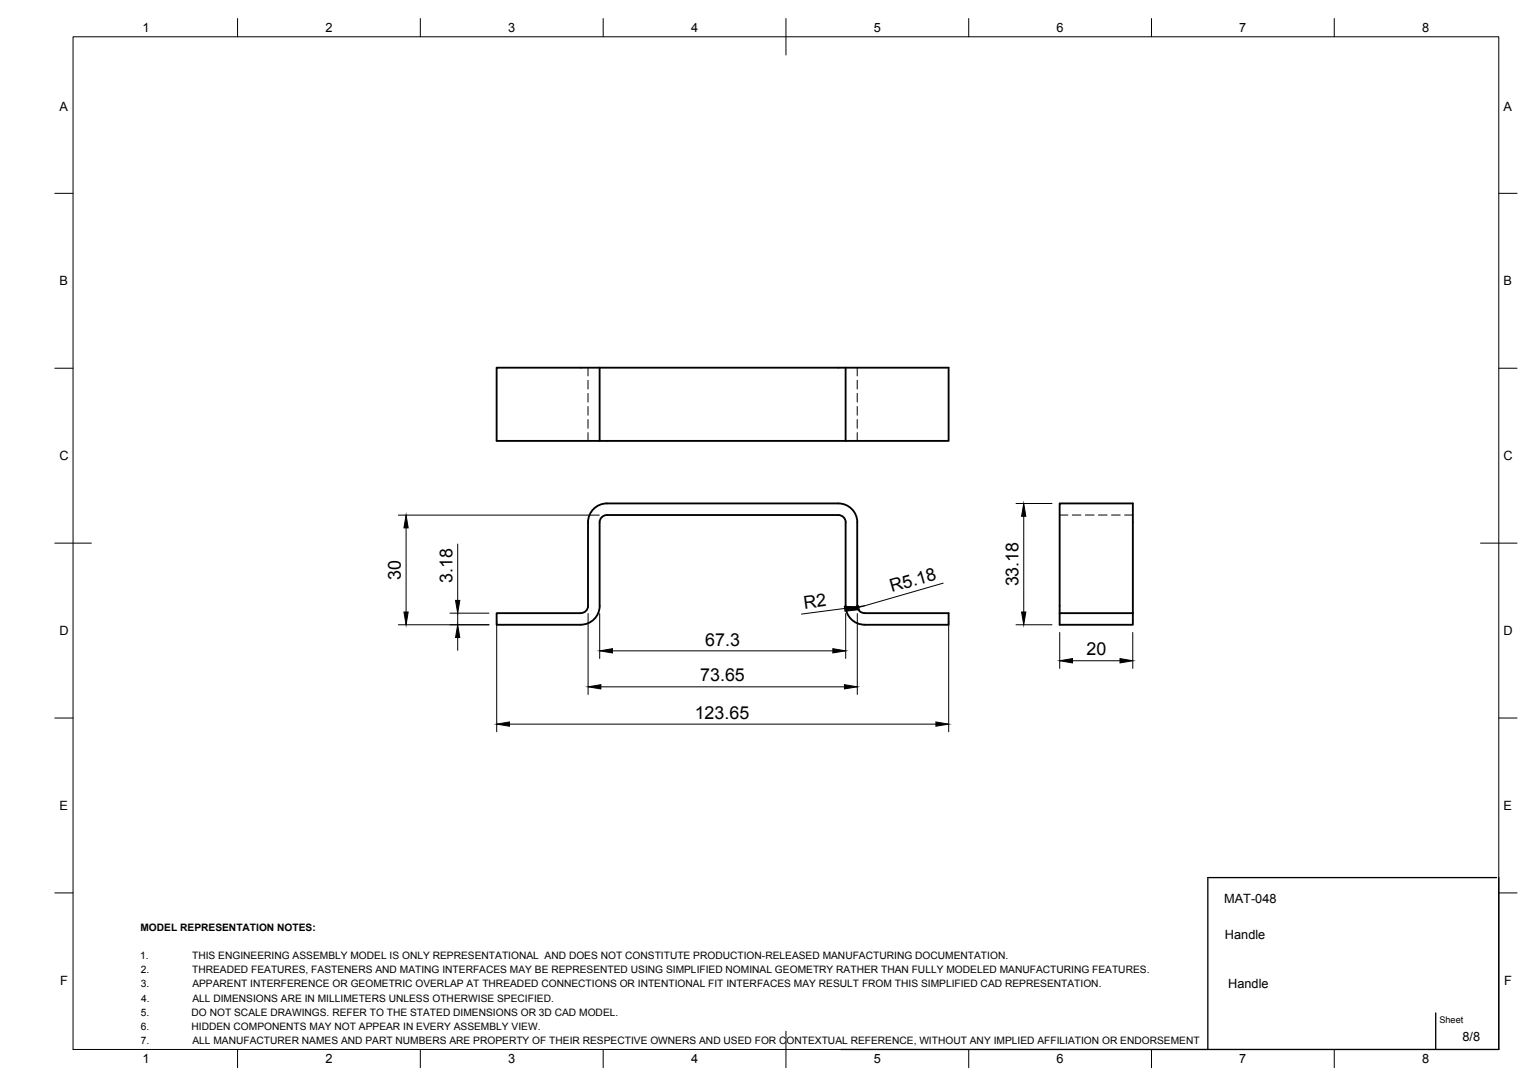
ISO-10303-21;
HEADER;
/* Generated by software containing ST-Developer
 * from STEP Tools, Inc. (www.steptools.com) 
 */

FILE_DESCRIPTION(
/* description */ ('STEP AP214'),
/* implementation_level */ '2;1');

FILE_NAME(
/* name */ 'Handle.step',
/* time_stamp */ '2026-11-14T22:24:45-08:00',
/* author */ (''),
/* organization */ (''),
/* preprocessor_version */ 'ST-DEVELOPER v20.2',
/* originating_system */ 'Autodesk Translation Framework v15.17.0.0',
/* authorisation */ '');

FILE_SCHEMA (('AUTOMOTIVE_DESIGN { 1 0 10303 214 3 1 1 }'));
ENDSEC;

DATA;
#10=MECHANICAL_DESIGN_GEOMETRIC_PRESENTATION_REPRESENTATION('',(#126),#5599);
#114=SHAPE_REPRESENTATION_RELATIONSHIP('SRR','None',#5642,#120);
#120=ADVANCED_BREP_SHAPE_REPRESENTATION('',(#132),#5594);
#126=STYLED_ITEM('',(#5681),#132);
#132=MANIFOLD_SOLID_BREP('Body1',#3308);
#157=CYLINDRICAL_SURFACE('',#3508,2.);
#158=CYLINDRICAL_SURFACE('',#3510,5.175);
#159=CYLINDRICAL_SURFACE('',#3512,5.175);
#160=CYLINDRICAL_SURFACE('',#3514,2.);
#161=CYLINDRICAL_SURFACE('',#3518,5.175);
#162=CYLINDRICAL_SURFACE('',#3520,2.);
#163=CYLINDRICAL_SURFACE('',#3522,2.);
#164=CYLINDRICAL_SURFACE('',#3524,5.175);
#209=CIRCLE('',#3474,2.);
#210=CIRCLE('',#3475,5.175);
#211=CIRCLE('',#3478,2.);
#212=CIRCLE('',#3479,5.175);
#213=CIRCLE('',#3482,5.175);
#214=CIRCLE('',#3483,2.);
#215=CIRCLE('',#3486,5.175);
#216=CIRCLE('',#3487,2.);
#217=CIRCLE('',#3490,5.175);
#218=CIRCLE('',#3491,2.);
#219=CIRCLE('',#3494,5.175);
#220=CIRCLE('',#3495,2.);
#221=CIRCLE('',#3498,2.);
#222=CIRCLE('',#3499,5.175);
#223=CIRCLE('',#3502,2.);
#224=CIRCLE('',#3503,5.175);
#347=FACE_OUTER_BOUND('',#523,.T.);
#348=FACE_OUTER_BOUND('',#524,.T.);
#349=FACE_OUTER_BOUND('',#525,.T.);
#350=FACE_OUTER_BOUND('',#526,.T.);
#351=FACE_OUTER_BOUND('',#527,.T.);
#352=FACE_OUTER_BOUND('',#528,.T.);
#353=FACE_OUTER_BOUND('',#529,.T.);
#354=FACE_OUTER_BOUND('',#530,.T.);
#355=FACE_OUTER_BOUND('',#531,.T.);
#356=FACE_OUTER_BOUND('',#532,.T.);
#357=FACE_OUTER_BOUND('',#533,.T.);
#358=FACE_OUTER_BOUND('',#534,.T.);
#359=FACE_OUTER_BOUND('',#535,.T.);
#360=FACE_OUTER_BOUND('',#536,.T.);
#361=FACE_OUTER_BOUND('',#537,.T.);
#362=FACE_OUTER_BOUND('',#538,.T.);
#363=FACE_OUTER_BOUND('',#539,.T.);
#364=FACE_OUTER_BOUND('',#540,.T.);
#365=FACE_OUTER_BOUND('',#541,.T.);
#366=FACE_OUTER_BOUND('',#542,.T.);
#367=FACE_OUTER_BOUND('',#543,.T.);
#368=FACE_OUTER_BOUND('',#544,.T.);
#369=FACE_OUTER_BOUND('',#545,.T.);
#370=FACE_OUTER_BOUND('',#546,.T.);
#371=FACE_OUTER_BOUND('',#547,.T.);
#372=FACE_OUTER_BOUND('',#548,.T.);
#373=FACE_OUTER_BOUND('',#549,.T.);
#374=FACE_OUTER_BOUND('',#550,.T.);
#375=FACE_OUTER_BOUND('',#551,.T.);
#376=FACE_OUTER_BOUND('',#552,.T.);
#377=FACE_OUTER_BOUND('',#553,.T.);
#378=FACE_OUTER_BOUND('',#554,.T.);
#379=FACE_OUTER_BOUND('',#555,.T.);
#380=FACE_OUTER_BOUND('',#556,.T.);
#381=FACE_OUTER_BOUND('',#557,.T.);
#382=FACE_OUTER_BOUND('',#558,.T.);
#383=FACE_OUTER_BOUND('',#559,.T.);
#384=FACE_OUTER_BOUND('',#560,.T.);
#523=EDGE_LOOP('',(#2483,#2484,#2485,#2486));
#524=EDGE_LOOP('',(#2487,#2488,#2489,#2490));
#525=EDGE_LOOP('',(#2491,#2492,#2493,#2494));
#526=EDGE_LOOP('',(#2495,#2496,#2497,#2498));
#527=EDGE_LOOP('',(#2499,#2500,#2501,#2502));
#528=EDGE_LOOP('',(#2503,#2504,#2505,#2506));
#529=EDGE_LOOP('',(#2507,#2508,#2509,#2510));
#530=EDGE_LOOP('',(#2511,#2512,#2513,#2514));
#531=EDGE_LOOP('',(#2515,#2516,#2517,#2518));
#532=EDGE_LOOP('',(#2519,#2520,#2521,#2522));
#533=EDGE_LOOP('',(#2523,#2524,#2525,#2526));
#534=EDGE_LOOP('',(#2527,#2528,#2529,#2530));
#535=EDGE_LOOP('',(#2531,#2532,#2533,#2534));
#536=EDGE_LOOP('',(#2535,#2536,#2537,#2538));
#537=EDGE_LOOP('',(#2539,#2540,#2541,#2542));
#538=EDGE_LOOP('',(#2543,#2544,#2545,#2546));
#539=EDGE_LOOP('',(#2547,#2548,#2549,#2550));
#540=EDGE_LOOP('',(#2551,#2552,#2553,#2554));
#541=EDGE_LOOP('',(#2555,#2556,#2557,#2558));
#542=EDGE_LOOP('',(#2559,#2560,#2561,#2562));
#543=EDGE_LOOP('',(#2563,#2564,#2565,#2566));
#544=EDGE_LOOP('',(#2567,#2568,#2569,#2570));
#545=EDGE_LOOP('',(#2571,#2572,#2573,#2574));
#546=EDGE_LOOP('',(#2575,#2576,#2577,#2578));
#547=EDGE_LOOP('',(#2579,#2580,#2581,#2582));
#548=EDGE_LOOP('',(#2583,#2584,#2585,#2586));
#549=EDGE_LOOP('',(#2587,#2588,#2589,#2590));
#550=EDGE_LOOP('',(#2591,#2592,#2593,#2594));
#551=EDGE_LOOP('',(#2595,#2596,#2597,#2598));
#552=EDGE_LOOP('',(#2599,#2600,#2601,#2602));
#553=EDGE_LOOP('',(#2603,#2604,#2605,#2606));
#554=EDGE_LOOP('',(#2607,#2608,#2609,#2610));
#555=EDGE_LOOP('',(#2611,#2612,#2613,#2614));
#556=EDGE_LOOP('',(#2615,#2616,#2617,#2618));
#557=EDGE_LOOP('',(#2619,#2620,#2621,#2622));
#558=EDGE_LOOP('',(#2623,#2624,#2625,#2626));
#559=EDGE_LOOP('',(#2627,#2628,#2629,#2630));
#560=EDGE_LOOP('',(#2631,#2632,#2633,#2634));
#815=LINE('',#5031,#1171);
#816=LINE('',#5035,#1172);
#817=LINE('',#5039,#1173);
#818=LINE('',#5041,#1174);
#819=LINE('',#5042,#1175);
#820=LINE('',#5046,#1176);
#821=LINE('',#5050,#1177);
#822=LINE('',#5054,#1178);
#823=LINE('',#5056,#1179);
#824=LINE('',#5057,#1180);
#825=LINE('',#5061,#1181);
#826=LINE('',#5066,#1182);
#827=LINE('',#5068,#1183);
#828=LINE('',#5069,#1184);
#829=LINE('',#5073,#1185);
#830=LINE('',#5077,#1186);
#831=LINE('',#5080,#1187);
#832=LINE('',#5081,#1188);
#833=LINE('',#5085,#1189);
#834=LINE('',#5090,#1190);
#835=LINE('',#5092,#1191);
#836=LINE('',#5093,#1192);
#837=LINE('',#5097,#1193);
#838=LINE('',#5101,#1194);
#839=LINE('',#5104,#1195);
#840=LINE('',#5105,#1196);
#841=LINE('',#5109,#1197);
#842=LINE('',#5114,#1198);
#843=LINE('',#5116,#1199);
#844=LINE('',#5117,#1200);
#845=LINE('',#5121,#1201);
#846=LINE('',#5125,#1202);
#847=LINE('',#5128,#1203);
#848=LINE('',#5129,#1204);
#849=LINE('',#5132,#1205);
#850=LINE('',#5133,#1206);
#851=LINE('',#5134,#1207);
#852=LINE('',#5137,#1208);
#853=LINE('',#5138,#1209);
#854=LINE('',#5140,#1210);
#855=LINE('',#5141,#1211);
#856=LINE('',#5143,#1212);
#857=LINE('',#5145,#1213);
#858=LINE('',#5147,#1214);
#859=LINE('',#5149,#1215);
#860=LINE('',#5151,#1216);
#861=LINE('',#5153,#1217);
#862=LINE('',#5155,#1218);
#863=LINE('',#5158,#1219);
#864=LINE('',#5159,#1220);
#865=LINE('',#5162,#1221);
#866=LINE('',#5163,#1222);
#867=LINE('',#5165,#1223);
#868=LINE('',#5166,#1224);
#869=LINE('',#5168,#1225);
#870=LINE('',#5170,#1226);
#871=LINE('',#5172,#1227);
#872=LINE('',#5174,#1228);
#873=LINE('',#5176,#1229);
#874=LINE('',#5178,#1230);
#1171=VECTOR('',#4037,1000.);
#1172=VECTOR('',#4040,1000.);
#1173=VECTOR('',#4045,1000.);
#1174=VECTOR('',#4046,1000.);
#1175=VECTOR('',#4047,1000.);
#1176=VECTOR('',#4050,1000.);
#1177=VECTOR('',#4053,1000.);
#1178=VECTOR('',#4058,1000.);
#1179=VECTOR('',#4059,1000.);
#1180=VECTOR('',#4060,1000.);
#1181=VECTOR('',#4063,1000.);
#1182=VECTOR('',#4070,1000.);
#1183=VECTOR('',#4071,1000.);
#1184=VECTOR('',#4072,1000.);
#1185=VECTOR('',#4075,1000.);
#1186=VECTOR('',#4078,1000.);
#1187=VECTOR('',#4083,1000.);
#1188=VECTOR('',#4084,1000.);
#1189=VECTOR('',#4087,1000.);
#1190=VECTOR('',#4094,1000.);
#1191=VECTOR('',#4095,1000.);
#1192=VECTOR('',#4096,1000.);
#1193=VECTOR('',#4099,1000.);
#1194=VECTOR('',#4102,1000.);
#1195=VECTOR('',#4107,1000.);
#1196=VECTOR('',#4108,1000.);
#1197=VECTOR('',#4111,1000.);
#1198=VECTOR('',#4118,1000.);
#1199=VECTOR('',#4119,1000.);
#1200=VECTOR('',#4120,1000.);
#1201=VECTOR('',#4123,1000.);
#1202=VECTOR('',#4126,1000.);
#1203=VECTOR('',#4131,1000.);
#1204=VECTOR('',#4132,1000.);
#1205=VECTOR('',#4135,1000.);
#1206=VECTOR('',#4136,1000.);
#1207=VECTOR('',#4137,1000.);
#1208=VECTOR('',#4140,1000.);
#1209=VECTOR('',#4141,1000.);
#1210=VECTOR('',#4144,1000.);
#1211=VECTOR('',#4145,1000.);
#1212=VECTOR('',#4148,1000.);
#1213=VECTOR('',#4151,1000.);
#1214=VECTOR('',#4154,1000.);
#1215=VECTOR('',#4157,1000.);
#1216=VECTOR('',#4160,1000.);
#1217=VECTOR('',#4163,1000.);
#1218=VECTOR('',#4166,1000.);
#1219=VECTOR('',#4169,1000.);
#1220=VECTOR('',#4170,1000.);
#1221=VECTOR('',#4173,1000.);
#1222=VECTOR('',#4174,1000.);
#1223=VECTOR('',#4177,1000.);
#1224=VECTOR('',#4178,1000.);
#1225=VECTOR('',#4181,1000.);
#1226=VECTOR('',#4184,1000.);
#1227=VECTOR('',#4187,1000.);
#1228=VECTOR('',#4190,1000.);
#1229=VECTOR('',#4193,1000.);
#1230=VECTOR('',#4196,1000.);
#1487=VERTEX_POINT('',#5029);
#1488=VERTEX_POINT('',#5030);
#1489=VERTEX_POINT('',#5032);
#1490=VERTEX_POINT('',#5034);
#1491=VERTEX_POINT('',#5038);
#1492=VERTEX_POINT('',#5040);
#1493=VERTEX_POINT('',#5044);
#1494=VERTEX_POINT('',#5045);
#1495=VERTEX_POINT('',#5047);
#1496=VERTEX_POINT('',#5049);
#1497=VERTEX_POINT('',#5053);
#1498=VERTEX_POINT('',#5055);
#1499=VERTEX_POINT('',#5059);
#1500=VERTEX_POINT('',#5060);
#1501=VERTEX_POINT('',#5065);
#1502=VERTEX_POINT('',#5067);
#1503=VERTEX_POINT('',#5071);
#1504=VERTEX_POINT('',#5072);
#1505=VERTEX_POINT('',#5074);
#1506=VERTEX_POINT('',#5076);
#1507=VERTEX_POINT('',#5083);
#1508=VERTEX_POINT('',#5084);
#1509=VERTEX_POINT('',#5089);
#1510=VERTEX_POINT('',#5091);
#1511=VERTEX_POINT('',#5095);
#1512=VERTEX_POINT('',#5096);
#1513=VERTEX_POINT('',#5098);
#1514=VERTEX_POINT('',#5100);
#1515=VERTEX_POINT('',#5107);
#1516=VERTEX_POINT('',#5108);
#1517=VERTEX_POINT('',#5113);
#1518=VERTEX_POINT('',#5115);
#1519=VERTEX_POINT('',#5119);
#1520=VERTEX_POINT('',#5120);
#1521=VERTEX_POINT('',#5122);
#1522=VERTEX_POINT('',#5124);
#1523=VERTEX_POINT('',#5131);
#1524=VERTEX_POINT('',#5136);
#1525=VERTEX_POINT('',#5157);
#1526=VERTEX_POINT('',#5161);
#1839=EDGE_CURVE('',#1487,#1488,#815,.T.);
#1840=EDGE_CURVE('',#1489,#1487,#209,.T.);
#1841=EDGE_CURVE('',#1490,#1489,#816,.T.);
#1842=EDGE_CURVE('',#1490,#1488,#210,.T.);
#1843=EDGE_CURVE('',#1487,#1491,#817,.T.);
#1844=EDGE_CURVE('',#1488,#1492,#818,.T.);
#1845=EDGE_CURVE('',#1492,#1491,#819,.T.);
#1846=EDGE_CURVE('',#1493,#1494,#820,.T.);
#1847=EDGE_CURVE('',#1493,#1495,#211,.T.);
#1848=EDGE_CURVE('',#1496,#1495,#821,.T.);
#1849=EDGE_CURVE('',#1494,#1496,#212,.T.);
#1850=EDGE_CURVE('',#1497,#1493,#822,.T.);
#1851=EDGE_CURVE('',#1498,#1494,#823,.T.);
#1852=EDGE_CURVE('',#1498,#1497,#824,.T.);
#1853=EDGE_CURVE('',#1499,#1500,#825,.T.);
#1854=EDGE_CURVE('',#1491,#1499,#213,.T.);
#1855=EDGE_CURVE('',#1492,#1500,#214,.T.);
#1856=EDGE_CURVE('',#1499,#1501,#826,.T.);
#1857=EDGE_CURVE('',#1500,#1502,#827,.T.);
#1858=EDGE_CURVE('',#1502,#1501,#828,.T.);
#1859=EDGE_CURVE('',#1503,#1504,#829,.T.);
#1860=EDGE_CURVE('',#1503,#1505,#215,.T.);
#1861=EDGE_CURVE('',#1506,#1505,#830,.T.);
#1862=EDGE_CURVE('',#1504,#1506,#216,.T.);
#1863=EDGE_CURVE('',#1495,#1503,#831,.T.);
#1864=EDGE_CURVE('',#1496,#1504,#832,.T.);
#1865=EDGE_CURVE('',#1507,#1508,#833,.T.);
#1866=EDGE_CURVE('',#1501,#1507,#217,.T.);
#1867=EDGE_CURVE('',#1502,#1508,#218,.T.);
#1868=EDGE_CURVE('',#1507,#1509,#834,.T.);
#1869=EDGE_CURVE('',#1508,#1510,#835,.T.);
#1870=EDGE_CURVE('',#1510,#1509,#836,.T.);
#1871=EDGE_CURVE('',#1511,#1512,#837,.T.);
#1872=EDGE_CURVE('',#1511,#1513,#219,.T.);
#1873=EDGE_CURVE('',#1514,#1513,#838,.T.);
#1874=EDGE_CURVE('',#1512,#1514,#220,.T.);
#1875=EDGE_CURVE('',#1505,#1511,#839,.T.);
#1876=EDGE_CURVE('',#1506,#1512,#840,.T.);
#1877=EDGE_CURVE('',#1515,#1516,#841,.T.);
#1878=EDGE_CURVE('',#1509,#1515,#221,.T.);
#1879=EDGE_CURVE('',#1510,#1516,#222,.T.);
#1880=EDGE_CURVE('',#1515,#1517,#842,.T.);
#1881=EDGE_CURVE('',#1516,#1518,#843,.T.);
#1882=EDGE_CURVE('',#1517,#1518,#844,.T.);
#1883=EDGE_CURVE('',#1519,#1520,#845,.T.);
#1884=EDGE_CURVE('',#1519,#1521,#223,.T.);
#1885=EDGE_CURVE('',#1522,#1521,#846,.T.);
#1886=EDGE_CURVE('',#1520,#1522,#224,.T.);
#1887=EDGE_CURVE('',#1513,#1519,#847,.T.);
#1888=EDGE_CURVE('',#1514,#1520,#848,.T.);
#1889=EDGE_CURVE('',#1522,#1523,#849,.T.);
#1890=EDGE_CURVE('',#1518,#1523,#850,.T.);
#1891=EDGE_CURVE('',#1516,#1522,#851,.T.);
#1892=EDGE_CURVE('',#1524,#1523,#852,.T.);
#1893=EDGE_CURVE('',#1517,#1524,#853,.T.);
#1894=EDGE_CURVE('',#1521,#1524,#854,.T.);
#1895=EDGE_CURVE('',#1515,#1521,#855,.T.);
#1896=EDGE_CURVE('',#1509,#1519,#856,.T.);
#1897=EDGE_CURVE('',#1507,#1513,#857,.T.);
#1898=EDGE_CURVE('',#1501,#1511,#858,.T.);
#1899=EDGE_CURVE('',#1499,#1505,#859,.T.);
#1900=EDGE_CURVE('',#1491,#1503,#860,.T.);
#1901=EDGE_CURVE('',#1487,#1495,#861,.T.);
#1902=EDGE_CURVE('',#1489,#1493,#862,.T.);
#1903=EDGE_CURVE('',#1525,#1497,#863,.T.);
#1904=EDGE_CURVE('',#1525,#1489,#864,.T.);
#1905=EDGE_CURVE('',#1526,#1498,#865,.T.);
#1906=EDGE_CURVE('',#1526,#1525,#866,.T.);
#1907=EDGE_CURVE('',#1490,#1494,#867,.T.);
#1908=EDGE_CURVE('',#1526,#1490,#868,.T.);
#1909=EDGE_CURVE('',#1488,#1496,#869,.T.);
#1910=EDGE_CURVE('',#1492,#1504,#870,.T.);
#1911=EDGE_CURVE('',#1500,#1506,#871,.T.);
#1912=EDGE_CURVE('',#1502,#1512,#872,.T.);
#1913=EDGE_CURVE('',#1508,#1514,#873,.T.);
#1914=EDGE_CURVE('',#1510,#1520,#874,.T.);
#2483=ORIENTED_EDGE('',*,*,#1839,.F.);
#2484=ORIENTED_EDGE('',*,*,#1840,.F.);
#2485=ORIENTED_EDGE('',*,*,#1841,.F.);
#2486=ORIENTED_EDGE('',*,*,#1842,.T.);
#2487=ORIENTED_EDGE('',*,*,#1843,.F.);
#2488=ORIENTED_EDGE('',*,*,#1839,.T.);
#2489=ORIENTED_EDGE('',*,*,#1844,.T.);
#2490=ORIENTED_EDGE('',*,*,#1845,.T.);
#2491=ORIENTED_EDGE('',*,*,#1846,.F.);
#2492=ORIENTED_EDGE('',*,*,#1847,.T.);
#2493=ORIENTED_EDGE('',*,*,#1848,.F.);
#2494=ORIENTED_EDGE('',*,*,#1849,.F.);
#2495=ORIENTED_EDGE('',*,*,#1850,.T.);
#2496=ORIENTED_EDGE('',*,*,#1846,.T.);
#2497=ORIENTED_EDGE('',*,*,#1851,.F.);
#2498=ORIENTED_EDGE('',*,*,#1852,.T.);
#2499=ORIENTED_EDGE('',*,*,#1853,.F.);
#2500=ORIENTED_EDGE('',*,*,#1854,.F.);
#2501=ORIENTED_EDGE('',*,*,#1845,.F.);
#2502=ORIENTED_EDGE('',*,*,#1855,.T.);
#2503=ORIENTED_EDGE('',*,*,#1856,.F.);
#2504=ORIENTED_EDGE('',*,*,#1853,.T.);
#2505=ORIENTED_EDGE('',*,*,#1857,.T.);
#2506=ORIENTED_EDGE('',*,*,#1858,.T.);
#2507=ORIENTED_EDGE('',*,*,#1859,.F.);
#2508=ORIENTED_EDGE('',*,*,#1860,.T.);
#2509=ORIENTED_EDGE('',*,*,#1861,.F.);
#2510=ORIENTED_EDGE('',*,*,#1862,.F.);
#2511=ORIENTED_EDGE('',*,*,#1863,.T.);
#2512=ORIENTED_EDGE('',*,*,#1859,.T.);
#2513=ORIENTED_EDGE('',*,*,#1864,.F.);
#2514=ORIENTED_EDGE('',*,*,#1848,.T.);
#2515=ORIENTED_EDGE('',*,*,#1865,.F.);
#2516=ORIENTED_EDGE('',*,*,#1866,.F.);
#2517=ORIENTED_EDGE('',*,*,#1858,.F.);
#2518=ORIENTED_EDGE('',*,*,#1867,.T.);
#2519=ORIENTED_EDGE('',*,*,#1868,.F.);
#2520=ORIENTED_EDGE('',*,*,#1865,.T.);
#2521=ORIENTED_EDGE('',*,*,#1869,.T.);
#2522=ORIENTED_EDGE('',*,*,#1870,.T.);
#2523=ORIENTED_EDGE('',*,*,#1871,.F.);
#2524=ORIENTED_EDGE('',*,*,#1872,.T.);
#2525=ORIENTED_EDGE('',*,*,#1873,.F.);
#2526=ORIENTED_EDGE('',*,*,#1874,.F.);
#2527=ORIENTED_EDGE('',*,*,#1875,.T.);
#2528=ORIENTED_EDGE('',*,*,#1871,.T.);
#2529=ORIENTED_EDGE('',*,*,#1876,.F.);
#2530=ORIENTED_EDGE('',*,*,#1861,.T.);
#2531=ORIENTED_EDGE('',*,*,#1877,.F.);
#2532=ORIENTED_EDGE('',*,*,#1878,.F.);
#2533=ORIENTED_EDGE('',*,*,#1870,.F.);
#2534=ORIENTED_EDGE('',*,*,#1879,.T.);
#2535=ORIENTED_EDGE('',*,*,#1880,.F.);
#2536=ORIENTED_EDGE('',*,*,#1877,.T.);
#2537=ORIENTED_EDGE('',*,*,#1881,.T.);
#2538=ORIENTED_EDGE('',*,*,#1882,.F.);
#2539=ORIENTED_EDGE('',*,*,#1883,.F.);
#2540=ORIENTED_EDGE('',*,*,#1884,.T.);
#2541=ORIENTED_EDGE('',*,*,#1885,.F.);
#2542=ORIENTED_EDGE('',*,*,#1886,.F.);
#2543=ORIENTED_EDGE('',*,*,#1887,.T.);
#2544=ORIENTED_EDGE('',*,*,#1883,.T.);
#2545=ORIENTED_EDGE('',*,*,#1888,.F.);
#2546=ORIENTED_EDGE('',*,*,#1873,.T.);
#2547=ORIENTED_EDGE('',*,*,#1889,.T.);
#2548=ORIENTED_EDGE('',*,*,#1890,.F.);
#2549=ORIENTED_EDGE('',*,*,#1881,.F.);
#2550=ORIENTED_EDGE('',*,*,#1891,.T.);
#2551=ORIENTED_EDGE('',*,*,#1892,.F.);
#2552=ORIENTED_EDGE('',*,*,#1893,.F.);
#2553=ORIENTED_EDGE('',*,*,#1882,.T.);
#2554=ORIENTED_EDGE('',*,*,#1890,.T.);
#2555=ORIENTED_EDGE('',*,*,#1894,.F.);
#2556=ORIENTED_EDGE('',*,*,#1895,.F.);
#2557=ORIENTED_EDGE('',*,*,#1880,.T.);
#2558=ORIENTED_EDGE('',*,*,#1893,.T.);
#2559=ORIENTED_EDGE('',*,*,#1884,.F.);
#2560=ORIENTED_EDGE('',*,*,#1896,.F.);
#2561=ORIENTED_EDGE('',*,*,#1878,.T.);
#2562=ORIENTED_EDGE('',*,*,#1895,.T.);
#2563=ORIENTED_EDGE('',*,*,#1887,.F.);
#2564=ORIENTED_EDGE('',*,*,#1897,.F.);
#2565=ORIENTED_EDGE('',*,*,#1868,.T.);
#2566=ORIENTED_EDGE('',*,*,#1896,.T.);
#2567=ORIENTED_EDGE('',*,*,#1872,.F.);
#2568=ORIENTED_EDGE('',*,*,#1898,.F.);
#2569=ORIENTED_EDGE('',*,*,#1866,.T.);
#2570=ORIENTED_EDGE('',*,*,#1897,.T.);
#2571=ORIENTED_EDGE('',*,*,#1875,.F.);
#2572=ORIENTED_EDGE('',*,*,#1899,.F.);
#2573=ORIENTED_EDGE('',*,*,#1856,.T.);
#2574=ORIENTED_EDGE('',*,*,#1898,.T.);
#2575=ORIENTED_EDGE('',*,*,#1860,.F.);
#2576=ORIENTED_EDGE('',*,*,#1900,.F.);
#2577=ORIENTED_EDGE('',*,*,#1854,.T.);
#2578=ORIENTED_EDGE('',*,*,#1899,.T.);
#2579=ORIENTED_EDGE('',*,*,#1863,.F.);
#2580=ORIENTED_EDGE('',*,*,#1901,.F.);
#2581=ORIENTED_EDGE('',*,*,#1843,.T.);
#2582=ORIENTED_EDGE('',*,*,#1900,.T.);
#2583=ORIENTED_EDGE('',*,*,#1847,.F.);
#2584=ORIENTED_EDGE('',*,*,#1902,.F.);
#2585=ORIENTED_EDGE('',*,*,#1840,.T.);
#2586=ORIENTED_EDGE('',*,*,#1901,.T.);
#2587=ORIENTED_EDGE('',*,*,#1850,.F.);
#2588=ORIENTED_EDGE('',*,*,#1903,.F.);
#2589=ORIENTED_EDGE('',*,*,#1904,.T.);
#2590=ORIENTED_EDGE('',*,*,#1902,.T.);
#2591=ORIENTED_EDGE('',*,*,#1852,.F.);
#2592=ORIENTED_EDGE('',*,*,#1905,.F.);
#2593=ORIENTED_EDGE('',*,*,#1906,.T.);
#2594=ORIENTED_EDGE('',*,*,#1903,.T.);
#2595=ORIENTED_EDGE('',*,*,#1851,.T.);
#2596=ORIENTED_EDGE('',*,*,#1907,.F.);
#2597=ORIENTED_EDGE('',*,*,#1908,.F.);
#2598=ORIENTED_EDGE('',*,*,#1905,.T.);
#2599=ORIENTED_EDGE('',*,*,#1849,.T.);
#2600=ORIENTED_EDGE('',*,*,#1909,.F.);
#2601=ORIENTED_EDGE('',*,*,#1842,.F.);
#2602=ORIENTED_EDGE('',*,*,#1907,.T.);
#2603=ORIENTED_EDGE('',*,*,#1864,.T.);
#2604=ORIENTED_EDGE('',*,*,#1910,.F.);
#2605=ORIENTED_EDGE('',*,*,#1844,.F.);
#2606=ORIENTED_EDGE('',*,*,#1909,.T.);
#2607=ORIENTED_EDGE('',*,*,#1862,.T.);
#2608=ORIENTED_EDGE('',*,*,#1911,.F.);
#2609=ORIENTED_EDGE('',*,*,#1855,.F.);
#2610=ORIENTED_EDGE('',*,*,#1910,.T.);
#2611=ORIENTED_EDGE('',*,*,#1876,.T.);
#2612=ORIENTED_EDGE('',*,*,#1912,.F.);
#2613=ORIENTED_EDGE('',*,*,#1857,.F.);
#2614=ORIENTED_EDGE('',*,*,#1911,.T.);
#2615=ORIENTED_EDGE('',*,*,#1874,.T.);
#2616=ORIENTED_EDGE('',*,*,#1913,.F.);
#2617=ORIENTED_EDGE('',*,*,#1867,.F.);
#2618=ORIENTED_EDGE('',*,*,#1912,.T.);
#2619=ORIENTED_EDGE('',*,*,#1888,.T.);
#2620=ORIENTED_EDGE('',*,*,#1914,.F.);
#2621=ORIENTED_EDGE('',*,*,#1869,.F.);
#2622=ORIENTED_EDGE('',*,*,#1913,.T.);
#2623=ORIENTED_EDGE('',*,*,#1886,.T.);
#2624=ORIENTED_EDGE('',*,*,#1891,.F.);
#2625=ORIENTED_EDGE('',*,*,#1879,.F.);
#2626=ORIENTED_EDGE('',*,*,#1914,.T.);
#2627=ORIENTED_EDGE('',*,*,#1908,.T.);
#2628=ORIENTED_EDGE('',*,*,#1841,.T.);
#2629=ORIENTED_EDGE('',*,*,#1904,.F.);
#2630=ORIENTED_EDGE('',*,*,#1906,.F.);
#2631=ORIENTED_EDGE('',*,*,#1889,.F.);
#2632=ORIENTED_EDGE('',*,*,#1885,.T.);
#2633=ORIENTED_EDGE('',*,*,#1894,.T.);
#2634=ORIENTED_EDGE('',*,*,#1892,.T.);
#3057=PLANE('',#3473);
#3058=PLANE('',#3476);
#3059=PLANE('',#3477);
#3060=PLANE('',#3480);
#3061=PLANE('',#3481);
#3062=PLANE('',#3484);
#3063=PLANE('',#3485);
#3064=PLANE('',#3488);
#3065=PLANE('',#3489);
#3066=PLANE('',#3492);
#3067=PLANE('',#3493);
#3068=PLANE('',#3496);
#3069=PLANE('',#3497);
#3070=PLANE('',#3500);
#3071=PLANE('',#3501);
#3072=PLANE('',#3504);
#3073=PLANE('',#3505);
#3074=PLANE('',#3506);
#3075=PLANE('',#3507);
#3076=PLANE('',#3509);
#3077=PLANE('',#3511);
#3078=PLANE('',#3513);
#3079=PLANE('',#3515);
#3080=PLANE('',#3516);
#3081=PLANE('',#3517);
#3082=PLANE('',#3519);
#3083=PLANE('',#3521);
#3084=PLANE('',#3523);
#3085=PLANE('',#3525);
#3086=PLANE('',#3526);
#3197=ADVANCED_FACE('',(#347),#3057,.T.);
#3198=ADVANCED_FACE('',(#348),#3058,.T.);
#3199=ADVANCED_FACE('',(#349),#3059,.T.);
#3200=ADVANCED_FACE('',(#350),#3060,.T.);
#3201=ADVANCED_FACE('',(#351),#3061,.T.);
#3202=ADVANCED_FACE('',(#352),#3062,.T.);
#3203=ADVANCED_FACE('',(#353),#3063,.T.);
#3204=ADVANCED_FACE('',(#354),#3064,.T.);
#3205=ADVANCED_FACE('',(#355),#3065,.T.);
#3206=ADVANCED_FACE('',(#356),#3066,.T.);
#3207=ADVANCED_FACE('',(#357),#3067,.T.);
#3208=ADVANCED_FACE('',(#358),#3068,.T.);
#3209=ADVANCED_FACE('',(#359),#3069,.T.);
#3210=ADVANCED_FACE('',(#360),#3070,.T.);
#3211=ADVANCED_FACE('',(#361),#3071,.T.);
#3212=ADVANCED_FACE('',(#362),#3072,.T.);
#3213=ADVANCED_FACE('',(#363),#3073,.F.);
#3214=ADVANCED_FACE('',(#364),#3074,.T.);
#3215=ADVANCED_FACE('',(#365),#3075,.T.);
#3216=ADVANCED_FACE('',(#366),#157,.F.);
#3217=ADVANCED_FACE('',(#367),#3076,.T.);
#3218=ADVANCED_FACE('',(#368),#158,.T.);
#3219=ADVANCED_FACE('',(#369),#3077,.T.);
#3220=ADVANCED_FACE('',(#370),#159,.T.);
#3221=ADVANCED_FACE('',(#371),#3078,.T.);
#3222=ADVANCED_FACE('',(#372),#160,.F.);
#3223=ADVANCED_FACE('',(#373),#3079,.T.);
#3224=ADVANCED_FACE('',(#374),#3080,.T.);
#3225=ADVANCED_FACE('',(#375),#3081,.F.);
#3226=ADVANCED_FACE('',(#376),#161,.T.);
#3227=ADVANCED_FACE('',(#377),#3082,.F.);
#3228=ADVANCED_FACE('',(#378),#162,.F.);
#3229=ADVANCED_FACE('',(#379),#3083,.F.);
#3230=ADVANCED_FACE('',(#380),#163,.F.);
#3231=ADVANCED_FACE('',(#381),#3084,.F.);
#3232=ADVANCED_FACE('',(#382),#164,.T.);
#3233=ADVANCED_FACE('',(#383),#3085,.F.);
#3234=ADVANCED_FACE('',(#384),#3086,.T.);
#3308=CLOSED_SHELL('',(#3197,#3198,#3199,#3200,#3201,#3202,#3203,#3204,
#3205,#3206,#3207,#3208,#3209,#3210,#3211,#3212,#3213,#3214,#3215,#3216,
#3217,#3218,#3219,#3220,#3221,#3222,#3223,#3224,#3225,#3226,#3227,#3228,
#3229,#3230,#3231,#3232,#3233,#3234));
#3472=AXIS2_PLACEMENT_3D('',#5027,#4033,#4034);
#3473=AXIS2_PLACEMENT_3D('',#5028,#4035,#4036);
#3474=AXIS2_PLACEMENT_3D('',#5033,#4038,#4039);
#3475=AXIS2_PLACEMENT_3D('',#5036,#4041,#4042);
#3476=AXIS2_PLACEMENT_3D('',#5037,#4043,#4044);
#3477=AXIS2_PLACEMENT_3D('',#5043,#4048,#4049);
#3478=AXIS2_PLACEMENT_3D('',#5048,#4051,#4052);
#3479=AXIS2_PLACEMENT_3D('',#5051,#4054,#4055);
#3480=AXIS2_PLACEMENT_3D('',#5052,#4056,#4057);
#3481=AXIS2_PLACEMENT_3D('',#5058,#4061,#4062);
#3482=AXIS2_PLACEMENT_3D('',#5062,#4064,#4065);
#3483=AXIS2_PLACEMENT_3D('',#5063,#4066,#4067);
#3484=AXIS2_PLACEMENT_3D('',#5064,#4068,#4069);
#3485=AXIS2_PLACEMENT_3D('',#5070,#4073,#4074);
#3486=AXIS2_PLACEMENT_3D('',#5075,#4076,#4077);
#3487=AXIS2_PLACEMENT_3D('',#5078,#4079,#4080);
#3488=AXIS2_PLACEMENT_3D('',#5079,#4081,#4082);
#3489=AXIS2_PLACEMENT_3D('',#5082,#4085,#4086);
#3490=AXIS2_PLACEMENT_3D('',#5086,#4088,#4089);
#3491=AXIS2_PLACEMENT_3D('',#5087,#4090,#4091);
#3492=AXIS2_PLACEMENT_3D('',#5088,#4092,#4093);
#3493=AXIS2_PLACEMENT_3D('',#5094,#4097,#4098);
#3494=AXIS2_PLACEMENT_3D('',#5099,#4100,#4101);
#3495=AXIS2_PLACEMENT_3D('',#5102,#4103,#4104);
#3496=AXIS2_PLACEMENT_3D('',#5103,#4105,#4106);
#3497=AXIS2_PLACEMENT_3D('',#5106,#4109,#4110);
#3498=AXIS2_PLACEMENT_3D('',#5110,#4112,#4113);
#3499=AXIS2_PLACEMENT_3D('',#5111,#4114,#4115);
#3500=AXIS2_PLACEMENT_3D('',#5112,#4116,#4117);
#3501=AXIS2_PLACEMENT_3D('',#5118,#4121,#4122);
#3502=AXIS2_PLACEMENT_3D('',#5123,#4124,#4125);
#3503=AXIS2_PLACEMENT_3D('',#5126,#4127,#4128);
#3504=AXIS2_PLACEMENT_3D('',#5127,#4129,#4130);
#3505=AXIS2_PLACEMENT_3D('',#5130,#4133,#4134);
#3506=AXIS2_PLACEMENT_3D('',#5135,#4138,#4139);
#3507=AXIS2_PLACEMENT_3D('',#5139,#4142,#4143);
#3508=AXIS2_PLACEMENT_3D('',#5142,#4146,#4147);
#3509=AXIS2_PLACEMENT_3D('',#5144,#4149,#4150);
#3510=AXIS2_PLACEMENT_3D('',#5146,#4152,#4153);
#3511=AXIS2_PLACEMENT_3D('',#5148,#4155,#4156);
#3512=AXIS2_PLACEMENT_3D('',#5150,#4158,#4159);
#3513=AXIS2_PLACEMENT_3D('',#5152,#4161,#4162);
#3514=AXIS2_PLACEMENT_3D('',#5154,#4164,#4165);
#3515=AXIS2_PLACEMENT_3D('',#5156,#4167,#4168);
#3516=AXIS2_PLACEMENT_3D('',#5160,#4171,#4172);
#3517=AXIS2_PLACEMENT_3D('',#5164,#4175,#4176);
#3518=AXIS2_PLACEMENT_3D('',#5167,#4179,#4180);
#3519=AXIS2_PLACEMENT_3D('',#5169,#4182,#4183);
#3520=AXIS2_PLACEMENT_3D('',#5171,#4185,#4186);
#3521=AXIS2_PLACEMENT_3D('',#5173,#4188,#4189);
#3522=AXIS2_PLACEMENT_3D('',#5175,#4191,#4192);
#3523=AXIS2_PLACEMENT_3D('',#5177,#4194,#4195);
#3524=AXIS2_PLACEMENT_3D('',#5179,#4197,#4198);
#3525=AXIS2_PLACEMENT_3D('',#5180,#4199,#4200);
#3526=AXIS2_PLACEMENT_3D('',#5181,#4201,#4202);
#4033=DIRECTION('axis',(0.,0.,1.));
#4034=DIRECTION('refdir',(1.,0.,0.));
#4035=DIRECTION('center_axis',(0.,0.,1.));
#4036=DIRECTION('ref_axis',(1.,0.,0.));
#4037=DIRECTION('',(1.,0.,0.));
#4038=DIRECTION('center_axis',(0.,0.,1.));
#4039=DIRECTION('ref_axis',(-1.,0.,0.));
#4040=DIRECTION('',(0.,1.,0.));
#4041=DIRECTION('center_axis',(0.,0.,1.));
#4042=DIRECTION('ref_axis',(1.,0.,0.));
#4043=DIRECTION('center_axis',(0.,0.,1.));
#4044=DIRECTION('ref_axis',(1.,0.,0.));
#4045=DIRECTION('',(0.,1.,0.));
#4046=DIRECTION('',(0.,1.,0.));
#4047=DIRECTION('',(-1.,0.,0.));
#4048=DIRECTION('center_axis',(0.,0.,-1.));
#4049=DIRECTION('ref_axis',(-1.,0.,0.));
#4050=DIRECTION('',(0.,-1.,0.));
#4051=DIRECTION('center_axis',(0.,0.,1.));
#4052=DIRECTION('ref_axis',(-1.,0.,0.));
#4053=DIRECTION('',(-1.,0.,0.));
#4054=DIRECTION('center_axis',(0.,0.,1.));
#4055=DIRECTION('ref_axis',(1.,0.,0.));
#4056=DIRECTION('center_axis',(0.,0.,-1.));
#4057=DIRECTION('ref_axis',(-1.,0.,0.));
#4058=DIRECTION('',(1.,0.,0.));
#4059=DIRECTION('',(1.,0.,0.));
#4060=DIRECTION('',(0.,1.,0.));
#4061=DIRECTION('center_axis',(0.,0.,1.));
#4062=DIRECTION('ref_axis',(1.,0.,0.));
#4063=DIRECTION('',(0.,-1.,0.));
#4064=DIRECTION('center_axis',(0.,0.,-1.));
#4065=DIRECTION('ref_axis',(1.,0.,0.));
#4066=DIRECTION('center_axis',(0.,0.,-1.));
#4067=DIRECTION('ref_axis',(1.,0.,0.));
#4068=DIRECTION('center_axis',(0.,0.,1.));
#4069=DIRECTION('ref_axis',(1.,0.,0.));
#4070=DIRECTION('',(1.,0.,0.));
#4071=DIRECTION('',(1.,0.,0.));
#4072=DIRECTION('',(0.,1.,0.));
#4073=DIRECTION('center_axis',(0.,0.,-1.));
#4074=DIRECTION('ref_axis',(-1.,0.,0.));
#4075=DIRECTION('',(1.,0.,0.));
#4076=DIRECTION('center_axis',(0.,0.,-1.));
#4077=DIRECTION('ref_axis',(1.,0.,0.));
#4078=DIRECTION('',(0.,1.,0.));
#4079=DIRECTION('center_axis',(0.,0.,-1.));
#4080=DIRECTION('ref_axis',(1.,0.,0.));
#4081=DIRECTION('center_axis',(0.,0.,-1.));
#4082=DIRECTION('ref_axis',(-1.,0.,0.));
#4083=DIRECTION('',(0.,1.,0.));
#4084=DIRECTION('',(0.,1.,0.));
#4085=DIRECTION('center_axis',(0.,0.,1.));
#4086=DIRECTION('ref_axis',(1.,0.,0.));
#4087=DIRECTION('',(-1.,0.,0.));
#4088=DIRECTION('center_axis',(0.,0.,-1.));
#4089=DIRECTION('ref_axis',(1.,0.,0.));
#4090=DIRECTION('center_axis',(0.,0.,-1.));
#4091=DIRECTION('ref_axis',(1.,0.,0.));
#4092=DIRECTION('center_axis',(0.,0.,1.));
#4093=DIRECTION('ref_axis',(1.,0.,0.));
#4094=DIRECTION('',(0.,-1.,0.));
#4095=DIRECTION('',(0.,-1.,0.));
#4096=DIRECTION('',(1.,-6.82961998416066E-16,0.));
#4097=DIRECTION('center_axis',(0.,0.,-1.));
#4098=DIRECTION('ref_axis',(-1.,0.,0.));
#4099=DIRECTION('',(0.,-1.,0.));
#4100=DIRECTION('center_axis',(0.,0.,-1.));
#4101=DIRECTION('ref_axis',(1.,0.,0.));
#4102=DIRECTION('',(1.,0.,0.));
#4103=DIRECTION('center_axis',(0.,0.,-1.));
#4104=DIRECTION('ref_axis',(1.,0.,0.));
#4105=DIRECTION('center_axis',(0.,0.,-1.));
#4106=DIRECTION('ref_axis',(-1.,0.,0.));
#4107=DIRECTION('',(1.,0.,0.));
#4108=DIRECTION('',(1.,0.,0.));
#4109=DIRECTION('center_axis',(0.,0.,1.));
#4110=DIRECTION('ref_axis',(1.,0.,0.));
#4111=DIRECTION('',(0.,-1.,0.));
#4112=DIRECTION('center_axis',(0.,0.,1.));
#4113=DIRECTION('ref_axis',(-1.,0.,0.));
#4114=DIRECTION('center_axis',(0.,0.,1.));
#4115=DIRECTION('ref_axis',(1.,0.,0.));
#4116=DIRECTION('center_axis',(0.,0.,1.));
#4117=DIRECTION('ref_axis',(1.,0.,0.));
#4118=DIRECTION('',(1.,0.,0.));
#4119=DIRECTION('',(1.,0.,0.));
#4120=DIRECTION('',(0.,-1.,0.));
#4121=DIRECTION('center_axis',(0.,0.,-1.));
#4122=DIRECTION('ref_axis',(-1.,0.,0.));
#4123=DIRECTION('',(-1.,6.82961998416066E-16,0.));
#4124=DIRECTION('center_axis',(0.,0.,1.));
#4125=DIRECTION('ref_axis',(-1.,0.,0.));
#4126=DIRECTION('',(0.,1.,0.));
#4127=DIRECTION('center_axis',(0.,0.,1.));
#4128=DIRECTION('ref_axis',(1.,0.,0.));
#4129=DIRECTION('center_axis',(0.,0.,-1.));
#4130=DIRECTION('ref_axis',(-1.,0.,0.));
#4131=DIRECTION('',(0.,-1.,0.));
#4132=DIRECTION('',(0.,-1.,0.));
#4133=DIRECTION('center_axis',(0.,1.,0.));
#4134=DIRECTION('ref_axis',(0.,0.,1.));
#4135=DIRECTION('',(1.,0.,0.));
#4136=DIRECTION('',(0.,0.,-1.));
#4137=DIRECTION('',(0.,0.,-1.));
#4138=DIRECTION('center_axis',(1.,0.,0.));
#4139=DIRECTION('ref_axis',(0.,0.,-1.));
#4140=DIRECTION('',(0.,-1.,0.));
#4141=DIRECTION('',(0.,0.,-1.));
#4142=DIRECTION('center_axis',(0.,1.,0.));
#4143=DIRECTION('ref_axis',(0.,0.,1.));
#4144=DIRECTION('',(1.,0.,0.));
#4145=DIRECTION('',(0.,0.,-1.));
#4146=DIRECTION('center_axis',(0.,0.,-1.));
#4147=DIRECTION('ref_axis',(-1.,0.,0.));
#4148=DIRECTION('',(0.,0.,-1.));
#4149=DIRECTION('center_axis',(1.,0.,0.));
#4150=DIRECTION('ref_axis',(0.,0.,-1.));
#4151=DIRECTION('',(0.,0.,-1.));
#4152=DIRECTION('center_axis',(0.,0.,-1.));
#4153=DIRECTION('ref_axis',(-1.,0.,0.));
#4154=DIRECTION('',(0.,0.,-1.));
#4155=DIRECTION('center_axis',(0.,1.,0.));
#4156=DIRECTION('ref_axis',(0.,0.,1.));
#4157=DIRECTION('',(0.,0.,-1.));
#4158=DIRECTION('center_axis',(0.,0.,-1.));
#4159=DIRECTION('ref_axis',(-1.,0.,0.));
#4160=DIRECTION('',(0.,0.,-1.));
#4161=DIRECTION('center_axis',(-1.,0.,0.));
#4162=DIRECTION('ref_axis',(0.,0.,1.));
#4163=DIRECTION('',(0.,0.,-1.));
#4164=DIRECTION('center_axis',(0.,0.,-1.));
#4165=DIRECTION('ref_axis',(-1.,0.,0.));
#4166=DIRECTION('',(0.,0.,-1.));
#4167=DIRECTION('center_axis',(0.,1.,0.));
#4168=DIRECTION('ref_axis',(0.,0.,1.));
#4169=DIRECTION('',(0.,0.,-1.));
#4170=DIRECTION('',(1.,0.,0.));
#4171=DIRECTION('center_axis',(-1.,0.,0.));
#4172=DIRECTION('ref_axis',(0.,0.,1.));
#4173=DIRECTION('',(0.,0.,-1.));
#4174=DIRECTION('',(0.,1.,0.));
#4175=DIRECTION('center_axis',(0.,1.,0.));
#4176=DIRECTION('ref_axis',(0.,0.,1.));
#4177=DIRECTION('',(0.,0.,-1.));
#4178=DIRECTION('',(1.,0.,0.));
#4179=DIRECTION('center_axis',(0.,0.,-1.));
#4180=DIRECTION('ref_axis',(-1.,0.,0.));
#4181=DIRECTION('',(0.,0.,-1.));
#4182=DIRECTION('center_axis',(-1.,0.,0.));
#4183=DIRECTION('ref_axis',(0.,0.,1.));
#4184=DIRECTION('',(0.,0.,-1.));
#4185=DIRECTION('center_axis',(0.,0.,-1.));
#4186=DIRECTION('ref_axis',(-1.,0.,0.));
#4187=DIRECTION('',(0.,0.,-1.));
#4188=DIRECTION('center_axis',(0.,1.,0.));
#4189=DIRECTION('ref_axis',(0.,0.,1.));
#4190=DIRECTION('',(0.,0.,-1.));
#4191=DIRECTION('center_axis',(0.,0.,-1.));
#4192=DIRECTION('ref_axis',(-1.,0.,0.));
#4193=DIRECTION('',(0.,0.,-1.));
#4194=DIRECTION('center_axis',(1.,0.,0.));
#4195=DIRECTION('ref_axis',(0.,0.,-1.));
#4196=DIRECTION('',(0.,0.,-1.));
#4197=DIRECTION('center_axis',(0.,0.,-1.));
#4198=DIRECTION('ref_axis',(-1.,0.,0.));
#4199=DIRECTION('center_axis',(0.,0.,-1.));
#4200=DIRECTION('ref_axis',(-1.,0.,0.));
#4201=DIRECTION('center_axis',(0.,0.,-1.));
#4202=DIRECTION('ref_axis',(-1.,0.,0.));
#5027=CARTESIAN_POINT('',(0.,0.,0.));
#5028=CARTESIAN_POINT('Origin',(25.,2.,20.));
#5029=CARTESIAN_POINT('',(25.,2.,20.));
#5030=CARTESIAN_POINT('',(28.175,2.,20.));
#5031=CARTESIAN_POINT('',(25.,2.,20.));
#5032=CARTESIAN_POINT('',(23.,0.,20.));
#5033=CARTESIAN_POINT('Origin',(23.,2.,20.));
#5034=CARTESIAN_POINT('',(23.,-3.17500000000001,20.));
#5035=CARTESIAN_POINT('',(23.,-3.17500000000001,20.));
#5036=CARTESIAN_POINT('Origin',(23.,2.,20.));
#5037=CARTESIAN_POINT('Origin',(23.,-3.17500000000001,20.));
#5038=CARTESIAN_POINT('',(25.,24.825,20.));
#5039=CARTESIAN_POINT('',(25.,0.,20.));
#5040=CARTESIAN_POINT('',(28.175,24.825,20.));
#5041=CARTESIAN_POINT('',(28.175,0.,20.));
#5042=CARTESIAN_POINT('',(28.175,24.825,20.));
#5043=CARTESIAN_POINT('Origin',(23.,0.,0.));
#5044=CARTESIAN_POINT('',(23.,0.,0.));
#5045=CARTESIAN_POINT('',(23.,-3.17500000000001,0.));
#5046=CARTESIAN_POINT('',(23.,0.,0.));
#5047=CARTESIAN_POINT('',(25.,2.,0.));
#5048=CARTESIAN_POINT('Origin',(23.,2.,0.));
#5049=CARTESIAN_POINT('',(28.175,2.,1.73472347597681E-15));
#5050=CARTESIAN_POINT('',(28.175,2.,1.73472347597681E-15));
#5051=CARTESIAN_POINT('Origin',(23.,2.,0.));
#5052=CARTESIAN_POINT('Origin',(28.175,2.,1.73472347597681E-15));
#5053=CARTESIAN_POINT('',(0.,0.,0.));
#5054=CARTESIAN_POINT('',(0.,0.,0.));
#5055=CARTESIAN_POINT('',(0.,-3.17500000000001,0.));
#5056=CARTESIAN_POINT('',(0.,-3.17500000000001,0.));
#5057=CARTESIAN_POINT('',(0.,-3.17500000000001,0.));
#5058=CARTESIAN_POINT('Origin',(30.175,30.,20.));
#5059=CARTESIAN_POINT('',(30.175,30.,20.));
#5060=CARTESIAN_POINT('',(30.175,26.825,20.));
#5061=CARTESIAN_POINT('',(30.175,30.,20.));
#5062=CARTESIAN_POINT('Origin',(30.175,24.825,20.));
#5063=CARTESIAN_POINT('Origin',(30.175,24.825,20.));
#5064=CARTESIAN_POINT('Origin',(28.175,24.825,20.));
#5065=CARTESIAN_POINT('',(93.4708296557372,30.,20.));
#5066=CARTESIAN_POINT('',(25.,30.,20.));
#5067=CARTESIAN_POINT('',(93.4708296557372,26.825,20.));
#5068=CARTESIAN_POINT('',(25.,26.825,20.));
#5069=CARTESIAN_POINT('',(93.4708296557372,26.825,20.));
#5070=CARTESIAN_POINT('Origin',(25.,24.825,0.));
#5071=CARTESIAN_POINT('',(25.,24.825,0.));
#5072=CARTESIAN_POINT('',(28.175,24.825,1.73472347597681E-15));
#5073=CARTESIAN_POINT('',(25.,24.825,0.));
#5074=CARTESIAN_POINT('',(30.175,30.,1.73472347597681E-15));
#5075=CARTESIAN_POINT('Origin',(30.175,24.825,1.73472347597681E-15));
#5076=CARTESIAN_POINT('',(30.175,26.825,1.73472347597681E-15));
#5077=CARTESIAN_POINT('',(30.175,26.825,1.73472347597681E-15));
#5078=CARTESIAN_POINT('Origin',(30.175,24.825,1.73472347597681E-15));
#5079=CARTESIAN_POINT('Origin',(30.175,26.825,1.73472347597681E-15));
#5080=CARTESIAN_POINT('',(25.,0.,0.));
#5081=CARTESIAN_POINT('',(28.175,0.,1.73472347597681E-15));
#5082=CARTESIAN_POINT('Origin',(98.6458296557372,24.825,20.));
#5083=CARTESIAN_POINT('',(98.6458296557372,24.825,20.));
#5084=CARTESIAN_POINT('',(95.4708296557372,24.825,20.));
#5085=CARTESIAN_POINT('',(98.6458296557372,24.825,20.));
#5086=CARTESIAN_POINT('Origin',(93.4708296557372,24.825,20.));
#5087=CARTESIAN_POINT('Origin',(93.4708296557372,24.825,20.));
#5088=CARTESIAN_POINT('Origin',(93.4708296557372,26.825,20.));
#5089=CARTESIAN_POINT('',(98.6458296557372,2.,20.));
#5090=CARTESIAN_POINT('',(98.6458296557372,30.,20.));
#5091=CARTESIAN_POINT('',(95.4708296557372,2.,20.));
#5092=CARTESIAN_POINT('',(95.4708296557372,30.,20.));
#5093=CARTESIAN_POINT('',(95.4708296557372,2.,20.));
#5094=CARTESIAN_POINT('Origin',(93.4708296557372,30.,1.73472347597681E-15));
#5095=CARTESIAN_POINT('',(93.4708296557372,30.,1.73472347597681E-15));
#5096=CARTESIAN_POINT('',(93.4708296557372,26.825,1.73472347597681E-15));
#5097=CARTESIAN_POINT('',(93.4708296557372,30.,1.73472347597681E-15));
#5098=CARTESIAN_POINT('',(98.6458296557372,24.825,0.));
#5099=CARTESIAN_POINT('Origin',(93.4708296557372,24.825,1.73472347597681E-15));
#5100=CARTESIAN_POINT('',(95.4708296557372,24.825,1.73472347597681E-15));
#5101=CARTESIAN_POINT('',(95.4708296557372,24.825,1.73472347597681E-15));
#5102=CARTESIAN_POINT('Origin',(93.4708296557372,24.825,1.73472347597681E-15));
#5103=CARTESIAN_POINT('Origin',(95.4708296557372,24.825,1.73472347597681E-15));
#5104=CARTESIAN_POINT('',(25.,30.,0.));
#5105=CARTESIAN_POINT('',(25.,26.825,0.));
#5106=CARTESIAN_POINT('Origin',(100.645829655737,0.,20.));
#5107=CARTESIAN_POINT('',(100.645829655737,0.,20.));
#5108=CARTESIAN_POINT('',(100.645829655737,-3.17500000000001,20.));
#5109=CARTESIAN_POINT('',(100.645829655737,0.,20.));
#5110=CARTESIAN_POINT('Origin',(100.645829655737,2.,20.));
#5111=CARTESIAN_POINT('Origin',(100.645829655737,2.,20.));
#5112=CARTESIAN_POINT('Origin',(95.4708296557372,2.,20.));
#5113=CARTESIAN_POINT('',(123.645829655737,0.,20.));
#5114=CARTESIAN_POINT('',(98.6458296557372,0.,20.));
#5115=CARTESIAN_POINT('',(123.645829655737,-3.17500000000001,20.));
#5116=CARTESIAN_POINT('',(98.6458296557372,-3.17500000000001,20.));
#5117=CARTESIAN_POINT('',(123.645829655737,0.,20.));
#5118=CARTESIAN_POINT('Origin',(98.6458296557372,2.,0.));
#5119=CARTESIAN_POINT('',(98.6458296557372,2.,0.));
#5120=CARTESIAN_POINT('',(95.4708296557372,2.,1.73472347597681E-15));
#5121=CARTESIAN_POINT('',(98.6458296557372,2.,0.));
#5122=CARTESIAN_POINT('',(100.645829655737,0.,0.));
#5123=CARTESIAN_POINT('Origin',(100.645829655737,2.,0.));
#5124=CARTESIAN_POINT('',(100.645829655737,-3.17500000000001,0.));
#5125=CARTESIAN_POINT('',(100.645829655737,-3.17500000000001,0.));
#5126=CARTESIAN_POINT('Origin',(100.645829655737,2.,0.));
#5127=CARTESIAN_POINT('Origin',(100.645829655737,-3.17500000000001,0.));
#5128=CARTESIAN_POINT('',(98.6458296557372,30.,0.));
#5129=CARTESIAN_POINT('',(95.4708296557372,30.,1.73472347597681E-15));
#5130=CARTESIAN_POINT('Origin',(98.6458296557372,-3.17500000000001,20.));
#5131=CARTESIAN_POINT('',(123.645829655737,-3.17500000000001,0.));
#5132=CARTESIAN_POINT('',(98.6458296557372,-3.17500000000001,0.));
#5133=CARTESIAN_POINT('',(123.645829655737,-3.17500000000001,20.));
#5134=CARTESIAN_POINT('',(100.645829655737,-3.17500000000001,20.));
#5135=CARTESIAN_POINT('Origin',(123.645829655737,0.,20.));
#5136=CARTESIAN_POINT('',(123.645829655737,0.,0.));
#5137=CARTESIAN_POINT('',(123.645829655737,0.,0.));
#5138=CARTESIAN_POINT('',(123.645829655737,0.,20.));
#5139=CARTESIAN_POINT('Origin',(98.6458296557372,0.,20.));
#5140=CARTESIAN_POINT('',(98.6458296557372,0.,0.));
#5141=CARTESIAN_POINT('',(100.645829655737,0.,20.));
#5142=CARTESIAN_POINT('Origin',(100.645829655737,2.,20.));
#5143=CARTESIAN_POINT('',(98.6458296557372,2.,20.));
#5144=CARTESIAN_POINT('Origin',(98.6458296557372,30.,20.));
#5145=CARTESIAN_POINT('',(98.6458296557372,24.825,20.));
#5146=CARTESIAN_POINT('Origin',(93.4708296557372,24.825,20.));
#5147=CARTESIAN_POINT('',(93.4708296557372,30.,20.));
#5148=CARTESIAN_POINT('Origin',(25.,30.,20.));
#5149=CARTESIAN_POINT('',(30.175,30.,20.));
#5150=CARTESIAN_POINT('Origin',(30.175,24.825,20.));
#5151=CARTESIAN_POINT('',(25.,24.825,20.));
#5152=CARTESIAN_POINT('Origin',(25.,0.,20.));
#5153=CARTESIAN_POINT('',(25.,2.,20.));
#5154=CARTESIAN_POINT('Origin',(23.,2.,20.));
#5155=CARTESIAN_POINT('',(23.,0.,20.));
#5156=CARTESIAN_POINT('Origin',(0.,0.,20.));
#5157=CARTESIAN_POINT('',(0.,0.,20.));
#5158=CARTESIAN_POINT('',(0.,0.,20.));
#5159=CARTESIAN_POINT('',(0.,0.,20.));
#5160=CARTESIAN_POINT('Origin',(0.,-3.17500000000001,20.));
#5161=CARTESIAN_POINT('',(0.,-3.17500000000001,20.));
#5162=CARTESIAN_POINT('',(0.,-3.17500000000001,20.));
#5163=CARTESIAN_POINT('',(0.,-3.17500000000001,20.));
#5164=CARTESIAN_POINT('Origin',(0.,-3.17500000000001,20.));
#5165=CARTESIAN_POINT('',(23.,-3.17500000000001,20.));
#5166=CARTESIAN_POINT('',(0.,-3.17500000000001,20.));
#5167=CARTESIAN_POINT('Origin',(23.,2.,20.));
#5168=CARTESIAN_POINT('',(28.175,2.,20.));
#5169=CARTESIAN_POINT('Origin',(28.175,0.,20.));
#5170=CARTESIAN_POINT('',(28.175,24.825,20.));
#5171=CARTESIAN_POINT('Origin',(30.175,24.825,20.));
#5172=CARTESIAN_POINT('',(30.175,26.825,20.));
#5173=CARTESIAN_POINT('Origin',(25.,26.825,20.));
#5174=CARTESIAN_POINT('',(93.4708296557372,26.825,20.));
#5175=CARTESIAN_POINT('Origin',(93.4708296557372,24.825,20.));
#5176=CARTESIAN_POINT('',(95.4708296557372,24.825,20.));
#5177=CARTESIAN_POINT('Origin',(95.4708296557372,30.,20.));
#5178=CARTESIAN_POINT('',(95.4708296557372,2.,20.));
#5179=CARTESIAN_POINT('Origin',(100.645829655737,2.,20.));
#5180=CARTESIAN_POINT('Origin',(100.645829655737,2.,20.));
#5181=CARTESIAN_POINT('Origin',(100.645829655737,2.,0.));
#5586=UNCERTAINTY_MEASURE_WITH_UNIT(LENGTH_MEASURE(0.01),#5600,
'DISTANCE_ACCURACY_VALUE',
'Maximum model space distance between geometric entities at asserted c
onnectivities');
#5591=UNCERTAINTY_MEASURE_WITH_UNIT(LENGTH_MEASURE(0.01),#5600,
'DISTANCE_ACCURACY_VALUE',
'Maximum model space distance between geometric entities at asserted c
onnectivities');
#5594=(
GEOMETRIC_REPRESENTATION_CONTEXT(3)
GLOBAL_UNCERTAINTY_ASSIGNED_CONTEXT((#5586))
GLOBAL_UNIT_ASSIGNED_CONTEXT((#5600,#5602,#5603))
REPRESENTATION_CONTEXT('','3D')
);
#5599=(
GEOMETRIC_REPRESENTATION_CONTEXT(3)
GLOBAL_UNCERTAINTY_ASSIGNED_CONTEXT((#5591))
GLOBAL_UNIT_ASSIGNED_CONTEXT((#5600,#5602,#5603))
REPRESENTATION_CONTEXT('','3D')
);
#5600=(
LENGTH_UNIT()
NAMED_UNIT(*)
SI_UNIT(.MILLI.,.METRE.)
);
#5602=(
NAMED_UNIT(*)
PLANE_ANGLE_UNIT()
SI_UNIT($,.RADIAN.)
);
#5603=(
NAMED_UNIT(*)
SI_UNIT($,.STERADIAN.)
SOLID_ANGLE_UNIT()
);
#5606=SHAPE_DEFINITION_REPRESENTATION(#5613,#5642);
#5613=PRODUCT_DEFINITION_SHAPE('',$,#5650);
#5642=SHAPE_REPRESENTATION('',(#3472),#5594);
#5647=PRODUCT_DEFINITION_CONTEXT('part definition',#5670,'design');
#5650=PRODUCT_DEFINITION('Handle','Handle',#5657,#5647);
#5657=PRODUCT_DEFINITION_FORMATION('',$,#5674);
#5670=APPLICATION_CONTEXT(
'Core Data for Automotive Mechanical Design Process');
#5671=PRODUCT_CONTEXT('part definition',#5670,'mechanical');
#5674=PRODUCT('Handle','Handle','Handle',(#5671));
#5681=PRESENTATION_STYLE_ASSIGNMENT((#5684));
#5684=SURFACE_STYLE_USAGE(.BOTH.,#5687);
#5687=SURFACE_SIDE_STYLE('',(#5690));
#5690=SURFACE_STYLE_FILL_AREA(#5693);
#5693=FILL_AREA_STYLE('Opaque(227,224,212)',(#5696));
#5696=FILL_AREA_STYLE_COLOUR('Opaque(227,224,212)',#5699);
#5699=COLOUR_RGB('Opaque(227,224,212)',0.890196078431372,0.87843137254902,
0.831372549019608);
ENDSEC;
END-ISO-10303-21;
